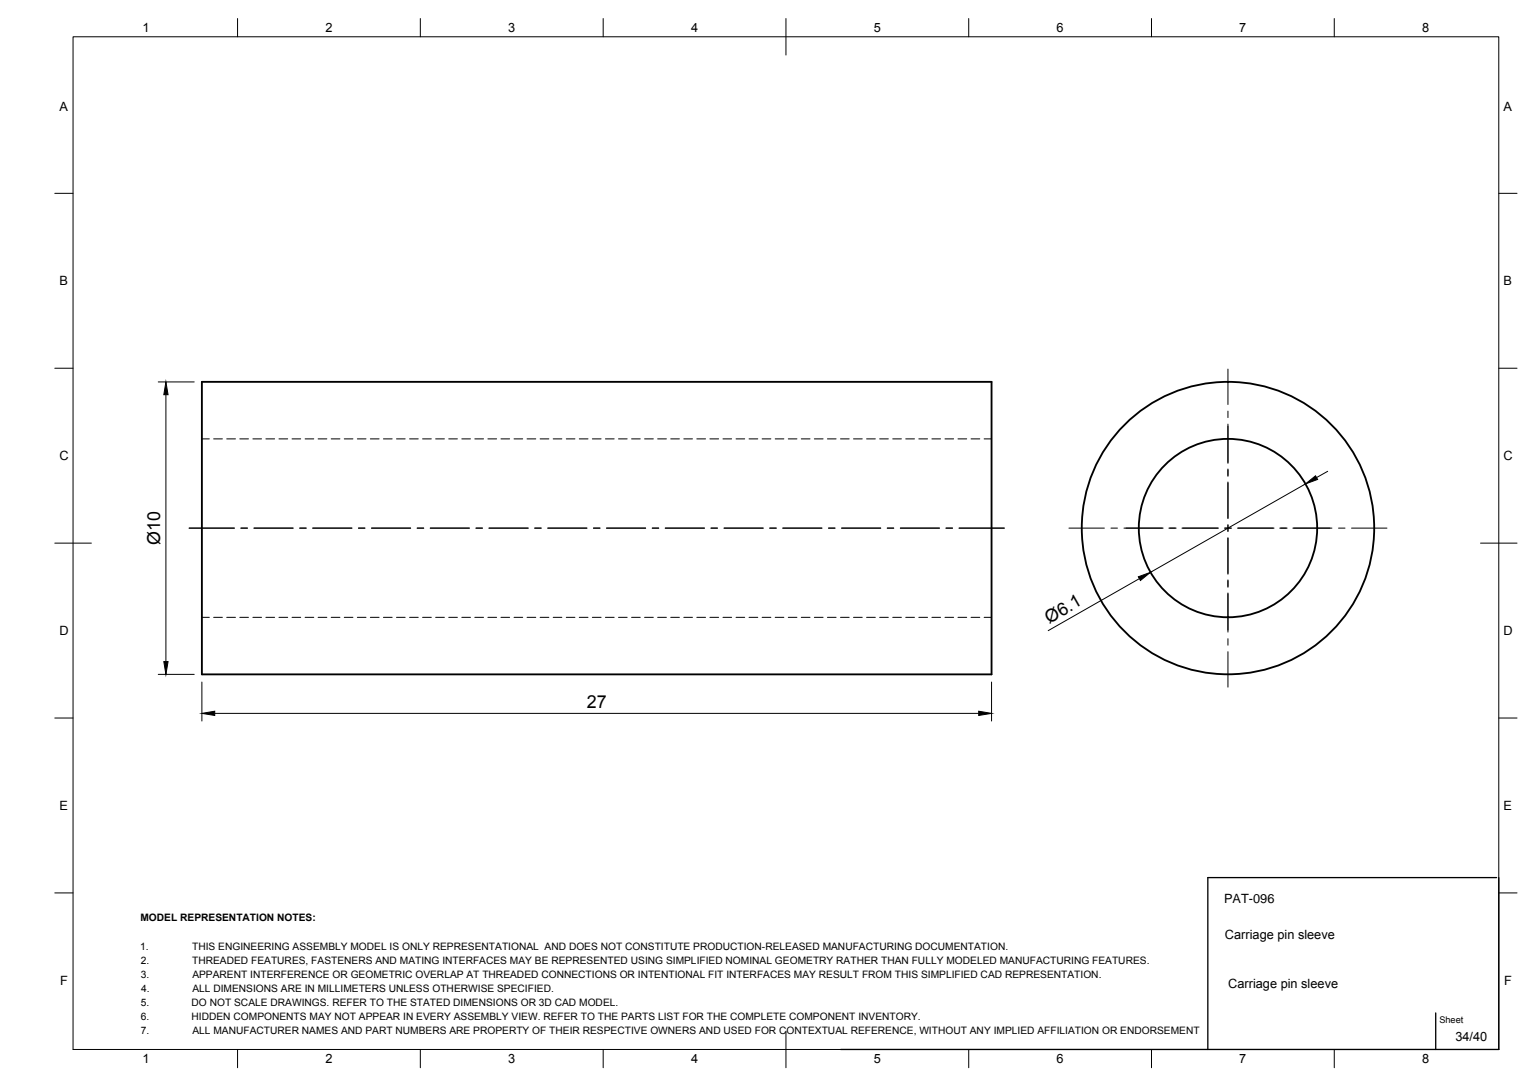
ISO-10303-21;
HEADER;
/* Generated by software containing ST-Developer
 * from STEP Tools, Inc. (www.steptools.com) 
 */

FILE_DESCRIPTION(
/* description */ ('PAT-096'),
/* implementation_level */ '2;1');

FILE_NAME(
/* name */ 'Carriage pin sleeve.step',
/* time_stamp */ '2026-10-29T17:03:14-07:00',
/* author */ (''),
/* organization */ (''),
/* preprocessor_version */ 'ST-DEVELOPER v20.2',
/* originating_system */ 'Autodesk Translation Framework v15.17.0.0',
/* authorisation */ '');

FILE_SCHEMA (('AUTOMOTIVE_DESIGN { 1 0 10303 214 3 1 1 }'));
ENDSEC;

DATA;
#10=MECHANICAL_DESIGN_GEOMETRIC_PRESENTATION_REPRESENTATION('',(#429),#10650);
#359=SHAPE_REPRESENTATION_RELATIONSHIP('SRR','None',#10823,#390);
#390=ADVANCED_BREP_SHAPE_REPRESENTATION('',(#466),#10641);
#429=STYLED_ITEM('',(#11064),#466);
#466=MANIFOLD_SOLID_BREP('Body1',#5564);
#573=FACE_BOUND('',#1488,.T.);
#574=FACE_BOUND('',#1490,.T.);
#743=PLANE('',#6474);
#744=PLANE('',#6475);
#1049=FACE_OUTER_BOUND('',#1485,.T.);
#1050=FACE_OUTER_BOUND('',#1486,.T.);
#1051=FACE_OUTER_BOUND('',#1487,.T.);
#1052=FACE_OUTER_BOUND('',#1489,.T.);
#1485=EDGE_LOOP('',(#4767,#4768,#4769,#4770));
#1486=EDGE_LOOP('',(#4771,#4772,#4773,#4774));
#1487=EDGE_LOOP('',(#4775));
#1488=EDGE_LOOP('',(#4776));
#1489=EDGE_LOOP('',(#4777));
#1490=EDGE_LOOP('',(#4778));
#1840=LINE('',#10183,#2169);
#1841=LINE('',#10189,#2170);
#2169=VECTOR('',#8020,0.305);
#2170=VECTOR('',#8027,0.5);
#2515=CIRCLE('',#6469,0.305);
#2516=CIRCLE('',#6470,0.305);
#2517=CIRCLE('',#6472,0.5);
#2518=CIRCLE('',#6473,0.5);
#2935=VERTEX_POINT('',#10180);
#2936=VERTEX_POINT('',#10182);
#2937=VERTEX_POINT('',#10186);
#2938=VERTEX_POINT('',#10188);
#3562=EDGE_CURVE('',#2935,#2935,#2515,.T.);
#3563=EDGE_CURVE('',#2935,#2936,#1840,.T.);
#3564=EDGE_CURVE('',#2936,#2936,#2516,.T.);
#3565=EDGE_CURVE('',#2937,#2937,#2517,.T.);
#3566=EDGE_CURVE('',#2937,#2938,#1841,.T.);
#3567=EDGE_CURVE('',#2938,#2938,#2518,.T.);
#4767=ORIENTED_EDGE('',*,*,#3562,.F.);
#4768=ORIENTED_EDGE('',*,*,#3563,.T.);
#4769=ORIENTED_EDGE('',*,*,#3564,.T.);
#4770=ORIENTED_EDGE('',*,*,#3563,.F.);
#4771=ORIENTED_EDGE('',*,*,#3565,.F.);
#4772=ORIENTED_EDGE('',*,*,#3566,.T.);
#4773=ORIENTED_EDGE('',*,*,#3567,.T.);
#4774=ORIENTED_EDGE('',*,*,#3566,.F.);
#4775=ORIENTED_EDGE('',*,*,#3565,.T.);
#4776=ORIENTED_EDGE('',*,*,#3562,.T.);
#4777=ORIENTED_EDGE('',*,*,#3567,.F.);
#4778=ORIENTED_EDGE('',*,*,#3564,.F.);
#5168=CYLINDRICAL_SURFACE('',#6468,0.305);
#5169=CYLINDRICAL_SURFACE('',#6471,0.5);
#5454=ADVANCED_FACE('',(#1049),#5168,.F.);
#5455=ADVANCED_FACE('',(#1050),#5169,.T.);
#5456=ADVANCED_FACE('',(#1051,#573),#743,.T.);
#5457=ADVANCED_FACE('',(#1052,#574),#744,.F.);
#5564=CLOSED_SHELL('',(#5454,#5455,#5456,#5457));
#6467=AXIS2_PLACEMENT_3D('',#10178,#8014,#8015);
#6468=AXIS2_PLACEMENT_3D('',#10179,#8016,#8017);
#6469=AXIS2_PLACEMENT_3D('',#10181,#8018,#8019);
#6470=AXIS2_PLACEMENT_3D('',#10184,#8021,#8022);
#6471=AXIS2_PLACEMENT_3D('',#10185,#8023,#8024);
#6472=AXIS2_PLACEMENT_3D('',#10187,#8025,#8026);
#6473=AXIS2_PLACEMENT_3D('',#10190,#8028,#8029);
#6474=AXIS2_PLACEMENT_3D('',#10191,#8030,#8031);
#6475=AXIS2_PLACEMENT_3D('',#10192,#8032,#8033);
#8014=DIRECTION('axis',(0.,0.,1.));
#8015=DIRECTION('refdir',(1.,0.,0.));
#8016=DIRECTION('center_axis',(0.,0.,1.));
#8017=DIRECTION('ref_axis',(1.,0.,0.));
#8018=DIRECTION('center_axis',(0.,0.,-1.));
#8019=DIRECTION('ref_axis',(1.,0.,0.));
#8020=DIRECTION('',(0.,0.,-1.));
#8021=DIRECTION('center_axis',(0.,0.,-1.));
#8022=DIRECTION('ref_axis',(1.,0.,0.));
#8023=DIRECTION('center_axis',(0.,0.,1.));
#8024=DIRECTION('ref_axis',(1.,0.,0.));
#8025=DIRECTION('center_axis',(0.,0.,1.));
#8026=DIRECTION('ref_axis',(1.,0.,0.));
#8027=DIRECTION('',(0.,0.,-1.));
#8028=DIRECTION('center_axis',(0.,0.,1.));
#8029=DIRECTION('ref_axis',(1.,0.,0.));
#8030=DIRECTION('center_axis',(0.,0.,1.));
#8031=DIRECTION('ref_axis',(1.,0.,0.));
#8032=DIRECTION('center_axis',(0.,0.,1.));
#8033=DIRECTION('ref_axis',(1.,0.,0.));
#10178=CARTESIAN_POINT('',(0.,0.,0.));
#10179=CARTESIAN_POINT('Origin',(7.5,4.,6.1));
#10180=CARTESIAN_POINT('',(7.195,4.,8.8));
#10181=CARTESIAN_POINT('Origin',(7.5,4.,8.8));
#10182=CARTESIAN_POINT('',(7.195,4.,6.1));
#10183=CARTESIAN_POINT('',(7.195,4.,6.1));
#10184=CARTESIAN_POINT('Origin',(7.5,4.,6.1));
#10185=CARTESIAN_POINT('Origin',(7.5,4.,6.1));
#10186=CARTESIAN_POINT('',(7.,4.,8.8));
#10187=CARTESIAN_POINT('Origin',(7.5,4.,8.8));
#10188=CARTESIAN_POINT('',(7.,4.,6.1));
#10189=CARTESIAN_POINT('',(7.,4.,6.1));
#10190=CARTESIAN_POINT('Origin',(7.5,4.,6.1));
#10191=CARTESIAN_POINT('Origin',(7.5,4.,8.8));
#10192=CARTESIAN_POINT('Origin',(7.5,4.,6.1));
#10602=UNCERTAINTY_MEASURE_WITH_UNIT(LENGTH_MEASURE(0.001),#10651,
'DISTANCE_ACCURACY_VALUE',
'Maximum model space distance between geometric entities at asserted c
onnectivities');
#10611=UNCERTAINTY_MEASURE_WITH_UNIT(LENGTH_MEASURE(0.001),#10651,
'DISTANCE_ACCURACY_VALUE',
'Maximum model space distance between geometric entities at asserted c
onnectivities');
#10641=(
GEOMETRIC_REPRESENTATION_CONTEXT(3)
GLOBAL_UNCERTAINTY_ASSIGNED_CONTEXT((#10602))
GLOBAL_UNIT_ASSIGNED_CONTEXT((#10651,#10653,#10654))
REPRESENTATION_CONTEXT('','3D')
);
#10650=(
GEOMETRIC_REPRESENTATION_CONTEXT(3)
GLOBAL_UNCERTAINTY_ASSIGNED_CONTEXT((#10611))
GLOBAL_UNIT_ASSIGNED_CONTEXT((#10651,#10653,#10654))
REPRESENTATION_CONTEXT('','3D')
);
#10651=(
LENGTH_UNIT()
NAMED_UNIT(*)
SI_UNIT(.CENTI.,.METRE.)
);
#10653=(
NAMED_UNIT(*)
PLANE_ANGLE_UNIT()
SI_UNIT($,.RADIAN.)
);
#10654=(
NAMED_UNIT(*)
SI_UNIT($,.STERADIAN.)
SOLID_ANGLE_UNIT()
);
#10684=SHAPE_DEFINITION_REPRESENTATION(#10730,#10823);
#10730=PRODUCT_DEFINITION_SHAPE('',$,#10862);
#10823=SHAPE_REPRESENTATION('',(#6467),#10641);
#10832=PRODUCT_DEFINITION_CONTEXT('part definition',#10948,'design');
#10862=PRODUCT_DEFINITION('Carriage pin sleeve','Carriage pin sleeve',#10900,
#10832);
#10900=PRODUCT_DEFINITION_FORMATION('',$,#10979);
#10948=APPLICATION_CONTEXT(
'Core Data for Automotive Mechanical Design Process');
#10949=PRODUCT_CONTEXT('part definition',#10948,'mechanical');
#10979=PRODUCT('Carriage pin sleeve','Carriage pin sleeve',
'Carriage pin sleeve',(#10949));
#11058=COLOUR_RGB('Grey',0.48,0.52,0.57);
#11059=FILL_AREA_STYLE_COLOUR('',#11058);
#11060=FILL_AREA_STYLE('',(#11059));
#11061=SURFACE_STYLE_FILL_AREA(#11060);
#11062=SURFACE_SIDE_STYLE('',(#11061));
#11063=SURFACE_STYLE_USAGE(.BOTH.,#11062);
#11064=PRESENTATION_STYLE_ASSIGNMENT((#11063));
ENDSEC;
END-ISO-10303-21;
